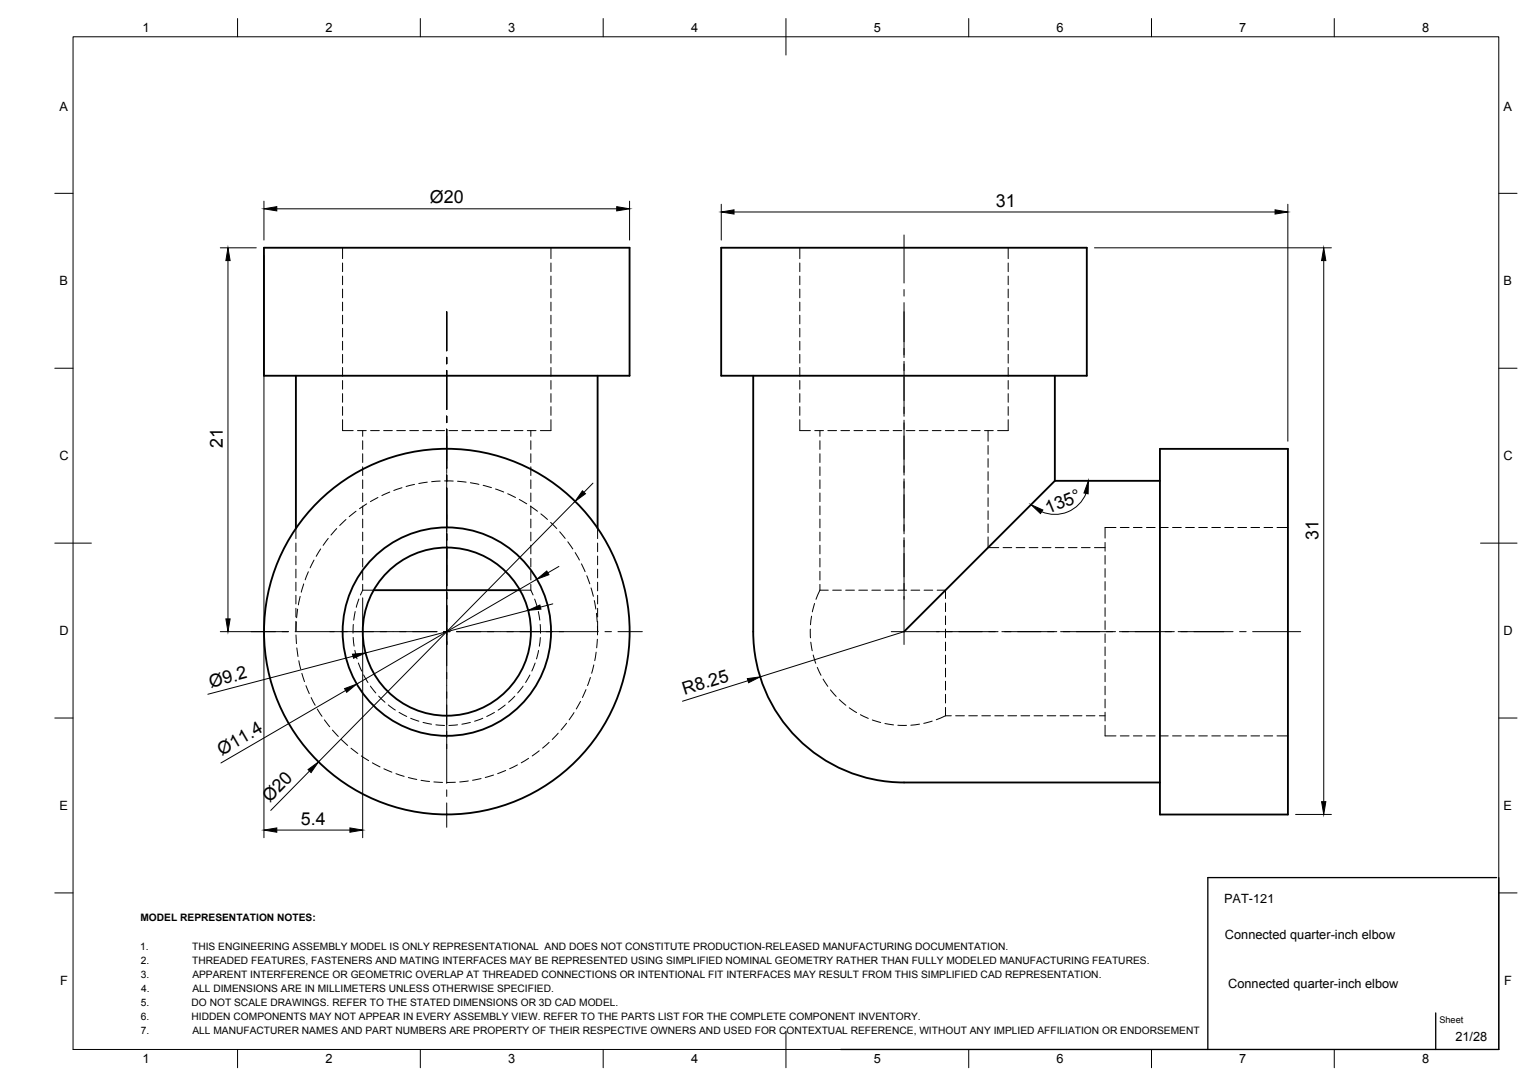
ISO-10303-21;
HEADER;
/* Generated by software containing ST-Developer
 * from STEP Tools, Inc. (www.steptools.com) 
 */

FILE_DESCRIPTION(
/* description */ ('Wall-mounted air drop station'),
/* implementation_level */ '2;1');

FILE_NAME(
/* name */ 'Connected quarter-inch elbow.step',
/* time_stamp */ '2026-10-28T22:16:19-07:00',
/* author */ (''),
/* organization */ (''),
/* preprocessor_version */ 'ST-DEVELOPER v20.2',
/* originating_system */ 'Autodesk Translation Framework v15.17.0.0',
/* authorisation */ '');

FILE_SCHEMA (('AUTOMOTIVE_DESIGN { 1 0 10303 214 3 1 1 }'));
ENDSEC;

DATA;
#10=MECHANICAL_DESIGN_GEOMETRIC_PRESENTATION_REPRESENTATION('',(#364),#10517);
#231=ELLIPSE('',#6687,0.650538238691624,0.46);
#232=ELLIPSE('',#6711,1.1667261889578,0.825);
#261=SPHERICAL_SURFACE('',#6691,0.513);
#262=SPHERICAL_SURFACE('',#6705,0.825);
#306=SHAPE_REPRESENTATION_RELATIONSHIP('SRR','None',#10663,#335);
#335=ADVANCED_BREP_SHAPE_REPRESENTATION('',(#391),#10507);
#364=STYLED_ITEM('',(#10888),#391);
#391=MANIFOLD_SOLID_BREP('Body1',#5905);
#505=FACE_BOUND('',#1465,.T.);
#506=FACE_BOUND('',#1468,.T.);
#507=FACE_BOUND('',#1472,.T.);
#508=FACE_BOUND('',#1476,.T.);
#509=FACE_BOUND('',#1479,.T.);
#510=FACE_BOUND('',#1481,.T.);
#511=FACE_BOUND('',#1484,.T.);
#676=PLANE('',#6697);
#677=PLANE('',#6704);
#678=PLANE('',#6713);
#679=PLANE('',#6717);
#680=PLANE('',#6718);
#681=PLANE('',#6723);
#1002=FACE_OUTER_BOUND('',#1463,.T.);
#1003=FACE_OUTER_BOUND('',#1464,.T.);
#1004=FACE_OUTER_BOUND('',#1466,.T.);
#1005=FACE_OUTER_BOUND('',#1467,.T.);
#1006=FACE_OUTER_BOUND('',#1469,.T.);
#1007=FACE_OUTER_BOUND('',#1470,.T.);
#1008=FACE_OUTER_BOUND('',#1471,.T.);
#1009=FACE_OUTER_BOUND('',#1473,.T.);
#1010=FACE_OUTER_BOUND('',#1474,.T.);
#1011=FACE_OUTER_BOUND('',#1475,.T.);
#1012=FACE_OUTER_BOUND('',#1477,.T.);
#1013=FACE_OUTER_BOUND('',#1478,.T.);
#1014=FACE_OUTER_BOUND('',#1480,.T.);
#1015=FACE_OUTER_BOUND('',#1482,.T.);
#1016=FACE_OUTER_BOUND('',#1483,.T.);
#1017=FACE_OUTER_BOUND('',#1485,.T.);
#1463=EDGE_LOOP('',(#4987,#4988,#4989,#4990,#4991,#4992));
#1464=EDGE_LOOP('',(#4993,#4994));
#1465=EDGE_LOOP('',(#4995,#4996,#4997,#4998));
#1466=EDGE_LOOP('',(#4999,#5000,#5001,#5002,#5003,#5004));
#1467=EDGE_LOOP('',(#5005));
#1468=EDGE_LOOP('',(#5006));
#1469=EDGE_LOOP('',(#5007,#5008,#5009,#5010));
#1470=EDGE_LOOP('',(#5011,#5012,#5013,#5014));
#1471=EDGE_LOOP('',(#5015));
#1472=EDGE_LOOP('',(#5016));
#1473=EDGE_LOOP('',(#5017,#5018,#5019,#5020));
#1474=EDGE_LOOP('',(#5021,#5022,#5023,#5024,#5025,#5026));
#1475=EDGE_LOOP('',(#5027));
#1476=EDGE_LOOP('',(#5028));
#1477=EDGE_LOOP('',(#5029,#5030,#5031,#5032));
#1478=EDGE_LOOP('',(#5033));
#1479=EDGE_LOOP('',(#5034));
#1480=EDGE_LOOP('',(#5035));
#1481=EDGE_LOOP('',(#5036));
#1482=EDGE_LOOP('',(#5037,#5038,#5039,#5040));
#1483=EDGE_LOOP('',(#5041));
#1484=EDGE_LOOP('',(#5042));
#1485=EDGE_LOOP('',(#5043,#5044,#5045,#5046,#5047,#5048));
#1906=LINE('',#9908,#2370);
#1907=LINE('',#9920,#2371);
#1908=LINE('',#9928,#2372);
#1909=LINE('',#9933,#2373);
#1910=LINE('',#9948,#2374);
#1911=LINE('',#9956,#2375);
#1912=LINE('',#9966,#2376);
#1913=LINE('',#9969,#2377);
#2370=VECTOR('',#8146,0.46);
#2371=VECTOR('',#8161,0.46);
#2372=VECTOR('',#8172,0.57);
#2373=VECTOR('',#8177,0.57);
#2374=VECTOR('',#8196,0.825);
#2375=VECTOR('',#8207,1.);
#2376=VECTOR('',#8220,1.);
#2377=VECTOR('',#8225,0.825);
#2701=CIRCLE('',#6688,0.46);
#2702=CIRCLE('',#6689,0.46);
#2703=CIRCLE('',#6690,0.46);
#2704=CIRCLE('',#6692,0.513);
#2705=CIRCLE('',#6693,0.46);
#2706=CIRCLE('',#6694,0.46);
#2707=CIRCLE('',#6696,0.46);
#2708=CIRCLE('',#6698,0.57);
#2709=CIRCLE('',#6700,0.57);
#2710=CIRCLE('',#6702,0.57);
#2711=CIRCLE('',#6703,0.57);
#2712=CIRCLE('',#6706,0.825);
#2713=CIRCLE('',#6707,0.825);
#2714=CIRCLE('',#6708,0.825);
#2715=CIRCLE('',#6709,0.825);
#2716=CIRCLE('',#6712,0.825);
#2717=CIRCLE('',#6714,1.);
#2718=CIRCLE('',#6716,1.);
#2719=CIRCLE('',#6719,1.);
#2720=CIRCLE('',#6720,0.825);
#2721=CIRCLE('',#6722,1.);
#3099=VERTEX_POINT('',#9902);
#3100=VERTEX_POINT('',#9903);
#3101=VERTEX_POINT('',#9905);
#3102=VERTEX_POINT('',#9907);
#3103=VERTEX_POINT('',#9912);
#3104=VERTEX_POINT('',#9913);
#3105=VERTEX_POINT('',#9915);
#3106=VERTEX_POINT('',#9919);
#3107=VERTEX_POINT('',#9923);
#3108=VERTEX_POINT('',#9926);
#3109=VERTEX_POINT('',#9930);
#3110=VERTEX_POINT('',#9932);
#3111=VERTEX_POINT('',#9937);
#3112=VERTEX_POINT('',#9938);
#3113=VERTEX_POINT('',#9940);
#3114=VERTEX_POINT('',#9942);
#3115=VERTEX_POINT('',#9947);
#3116=VERTEX_POINT('',#9951);
#3117=VERTEX_POINT('',#9954);
#3118=VERTEX_POINT('',#9959);
#3119=VERTEX_POINT('',#9961);
#3120=VERTEX_POINT('',#9964);
#3751=EDGE_CURVE('',#3099,#3100,#231,.T.);
#3752=EDGE_CURVE('',#3101,#3099,#2701,.T.);
#3753=EDGE_CURVE('',#3101,#3102,#1906,.T.);
#3754=EDGE_CURVE('',#3102,#3102,#2702,.T.);
#3755=EDGE_CURVE('',#3100,#3101,#2703,.T.);
#3756=EDGE_CURVE('',#3103,#3104,#2704,.T.);
#3757=EDGE_CURVE('',#3099,#3105,#2705,.T.);
#3758=EDGE_CURVE('',#3105,#3100,#2706,.T.);
#3759=EDGE_CURVE('',#3105,#3106,#1907,.T.);
#3760=EDGE_CURVE('',#3106,#3106,#2707,.T.);
#3761=EDGE_CURVE('',#3107,#3107,#2708,.T.);
#3762=EDGE_CURVE('',#3108,#3108,#2709,.T.);
#3763=EDGE_CURVE('',#3108,#3107,#1908,.T.);
#3764=EDGE_CURVE('',#3109,#3109,#2710,.T.);
#3765=EDGE_CURVE('',#3109,#3110,#1909,.T.);
#3766=EDGE_CURVE('',#3110,#3110,#2711,.T.);
#3767=EDGE_CURVE('',#3111,#3112,#2712,.T.);
#3768=EDGE_CURVE('',#3112,#3113,#2713,.T.);
#3769=EDGE_CURVE('',#3114,#3113,#2714,.T.);
#3770=EDGE_CURVE('',#3111,#3114,#2715,.T.);
#3771=EDGE_CURVE('',#3113,#3111,#232,.T.);
#3772=EDGE_CURVE('',#3112,#3115,#1910,.T.);
#3773=EDGE_CURVE('',#3115,#3115,#2716,.T.);
#3774=EDGE_CURVE('',#3116,#3116,#2717,.T.);
#3775=EDGE_CURVE('',#3117,#3117,#2718,.T.);
#3776=EDGE_CURVE('',#3117,#3116,#1911,.T.);
#3777=EDGE_CURVE('',#3118,#3118,#2719,.T.);
#3778=EDGE_CURVE('',#3119,#3119,#2720,.T.);
#3779=EDGE_CURVE('',#3120,#3120,#2721,.T.);
#3780=EDGE_CURVE('',#3120,#3118,#1912,.T.);
#3781=EDGE_CURVE('',#3119,#3114,#1913,.T.);
#4987=ORIENTED_EDGE('',*,*,#3751,.F.);
#4988=ORIENTED_EDGE('',*,*,#3752,.F.);
#4989=ORIENTED_EDGE('',*,*,#3753,.T.);
#4990=ORIENTED_EDGE('',*,*,#3754,.F.);
#4991=ORIENTED_EDGE('',*,*,#3753,.F.);
#4992=ORIENTED_EDGE('',*,*,#3755,.F.);
#4993=ORIENTED_EDGE('',*,*,#3756,.T.);
#4994=ORIENTED_EDGE('',*,*,#3756,.F.);
#4995=ORIENTED_EDGE('',*,*,#3755,.T.);
#4996=ORIENTED_EDGE('',*,*,#3752,.T.);
#4997=ORIENTED_EDGE('',*,*,#3757,.T.);
#4998=ORIENTED_EDGE('',*,*,#3758,.T.);
#4999=ORIENTED_EDGE('',*,*,#3751,.T.);
#5000=ORIENTED_EDGE('',*,*,#3758,.F.);
#5001=ORIENTED_EDGE('',*,*,#3759,.T.);
#5002=ORIENTED_EDGE('',*,*,#3760,.F.);
#5003=ORIENTED_EDGE('',*,*,#3759,.F.);
#5004=ORIENTED_EDGE('',*,*,#3757,.F.);
#5005=ORIENTED_EDGE('',*,*,#3761,.F.);
#5006=ORIENTED_EDGE('',*,*,#3754,.T.);
#5007=ORIENTED_EDGE('',*,*,#3762,.F.);
#5008=ORIENTED_EDGE('',*,*,#3763,.T.);
#5009=ORIENTED_EDGE('',*,*,#3761,.T.);
#5010=ORIENTED_EDGE('',*,*,#3763,.F.);
#5011=ORIENTED_EDGE('',*,*,#3764,.F.);
#5012=ORIENTED_EDGE('',*,*,#3765,.T.);
#5013=ORIENTED_EDGE('',*,*,#3766,.F.);
#5014=ORIENTED_EDGE('',*,*,#3765,.F.);
#5015=ORIENTED_EDGE('',*,*,#3764,.T.);
#5016=ORIENTED_EDGE('',*,*,#3760,.T.);
#5017=ORIENTED_EDGE('',*,*,#3767,.T.);
#5018=ORIENTED_EDGE('',*,*,#3768,.T.);
#5019=ORIENTED_EDGE('',*,*,#3769,.F.);
#5020=ORIENTED_EDGE('',*,*,#3770,.F.);
#5021=ORIENTED_EDGE('',*,*,#3771,.F.);
#5022=ORIENTED_EDGE('',*,*,#3768,.F.);
#5023=ORIENTED_EDGE('',*,*,#3772,.T.);
#5024=ORIENTED_EDGE('',*,*,#3773,.T.);
#5025=ORIENTED_EDGE('',*,*,#3772,.F.);
#5026=ORIENTED_EDGE('',*,*,#3767,.F.);
#5027=ORIENTED_EDGE('',*,*,#3774,.F.);
#5028=ORIENTED_EDGE('',*,*,#3762,.T.);
#5029=ORIENTED_EDGE('',*,*,#3775,.F.);
#5030=ORIENTED_EDGE('',*,*,#3776,.T.);
#5031=ORIENTED_EDGE('',*,*,#3774,.T.);
#5032=ORIENTED_EDGE('',*,*,#3776,.F.);
#5033=ORIENTED_EDGE('',*,*,#3775,.T.);
#5034=ORIENTED_EDGE('',*,*,#3773,.F.);
#5035=ORIENTED_EDGE('',*,*,#3777,.F.);
#5036=ORIENTED_EDGE('',*,*,#3778,.T.);
#5037=ORIENTED_EDGE('',*,*,#3779,.F.);
#5038=ORIENTED_EDGE('',*,*,#3780,.T.);
#5039=ORIENTED_EDGE('',*,*,#3777,.T.);
#5040=ORIENTED_EDGE('',*,*,#3780,.F.);
#5041=ORIENTED_EDGE('',*,*,#3779,.T.);
#5042=ORIENTED_EDGE('',*,*,#3766,.T.);
#5043=ORIENTED_EDGE('',*,*,#3778,.F.);
#5044=ORIENTED_EDGE('',*,*,#3781,.T.);
#5045=ORIENTED_EDGE('',*,*,#3769,.T.);
#5046=ORIENTED_EDGE('',*,*,#3771,.T.);
#5047=ORIENTED_EDGE('',*,*,#3770,.T.);
#5048=ORIENTED_EDGE('',*,*,#3781,.F.);
#5509=CYLINDRICAL_SURFACE('',#6686,0.46);
#5510=CYLINDRICAL_SURFACE('',#6695,0.46);
#5511=CYLINDRICAL_SURFACE('',#6699,0.57);
#5512=CYLINDRICAL_SURFACE('',#6701,0.57);
#5513=CYLINDRICAL_SURFACE('',#6710,0.825);
#5514=CYLINDRICAL_SURFACE('',#6715,1.);
#5515=CYLINDRICAL_SURFACE('',#6721,1.);
#5516=CYLINDRICAL_SURFACE('',#6724,0.825);
#5775=ADVANCED_FACE('',(#1002),#5509,.F.);
#5776=ADVANCED_FACE('',(#1003,#505),#261,.F.);
#5777=ADVANCED_FACE('',(#1004),#5510,.F.);
#5778=ADVANCED_FACE('',(#1005,#506),#676,.F.);
#5779=ADVANCED_FACE('',(#1006),#5511,.F.);
#5780=ADVANCED_FACE('',(#1007),#5512,.F.);
#5781=ADVANCED_FACE('',(#1008,#507),#677,.F.);
#5782=ADVANCED_FACE('',(#1009),#262,.T.);
#5783=ADVANCED_FACE('',(#1010),#5513,.T.);
#5784=ADVANCED_FACE('',(#1011,#508),#678,.T.);
#5785=ADVANCED_FACE('',(#1012),#5514,.T.);
#5786=ADVANCED_FACE('',(#1013,#509),#679,.T.);
#5787=ADVANCED_FACE('',(#1014,#510),#680,.T.);
#5788=ADVANCED_FACE('',(#1015),#5515,.T.);
#5789=ADVANCED_FACE('',(#1016,#511),#681,.T.);
#5790=ADVANCED_FACE('',(#1017),#5516,.T.);
#5905=CLOSED_SHELL('',(#5775,#5776,#5777,#5778,#5779,#5780,#5781,#5782,
#5783,#5784,#5785,#5786,#5787,#5788,#5789,#5790));
#6685=AXIS2_PLACEMENT_3D('',#9900,#8138,#8139);
#6686=AXIS2_PLACEMENT_3D('',#9901,#8140,#8141);
#6687=AXIS2_PLACEMENT_3D('',#9904,#8142,#8143);
#6688=AXIS2_PLACEMENT_3D('',#9906,#8144,#8145);
#6689=AXIS2_PLACEMENT_3D('',#9909,#8147,#8148);
#6690=AXIS2_PLACEMENT_3D('',#9910,#8149,#8150);
#6691=AXIS2_PLACEMENT_3D('',#9911,#8151,#8152);
#6692=AXIS2_PLACEMENT_3D('',#9914,#8153,#8154);
#6693=AXIS2_PLACEMENT_3D('',#9916,#8155,#8156);
#6694=AXIS2_PLACEMENT_3D('',#9917,#8157,#8158);
#6695=AXIS2_PLACEMENT_3D('',#9918,#8159,#8160);
#6696=AXIS2_PLACEMENT_3D('',#9921,#8162,#8163);
#6697=AXIS2_PLACEMENT_3D('',#9922,#8164,#8165);
#6698=AXIS2_PLACEMENT_3D('',#9924,#8166,#8167);
#6699=AXIS2_PLACEMENT_3D('',#9925,#8168,#8169);
#6700=AXIS2_PLACEMENT_3D('',#9927,#8170,#8171);
#6701=AXIS2_PLACEMENT_3D('',#9929,#8173,#8174);
#6702=AXIS2_PLACEMENT_3D('',#9931,#8175,#8176);
#6703=AXIS2_PLACEMENT_3D('',#9934,#8178,#8179);
#6704=AXIS2_PLACEMENT_3D('',#9935,#8180,#8181);
#6705=AXIS2_PLACEMENT_3D('',#9936,#8182,#8183);
#6706=AXIS2_PLACEMENT_3D('',#9939,#8184,#8185);
#6707=AXIS2_PLACEMENT_3D('',#9941,#8186,#8187);
#6708=AXIS2_PLACEMENT_3D('',#9943,#8188,#8189);
#6709=AXIS2_PLACEMENT_3D('',#9944,#8190,#8191);
#6710=AXIS2_PLACEMENT_3D('',#9945,#8192,#8193);
#6711=AXIS2_PLACEMENT_3D('',#9946,#8194,#8195);
#6712=AXIS2_PLACEMENT_3D('',#9949,#8197,#8198);
#6713=AXIS2_PLACEMENT_3D('',#9950,#8199,#8200);
#6714=AXIS2_PLACEMENT_3D('',#9952,#8201,#8202);
#6715=AXIS2_PLACEMENT_3D('',#9953,#8203,#8204);
#6716=AXIS2_PLACEMENT_3D('',#9955,#8205,#8206);
#6717=AXIS2_PLACEMENT_3D('',#9957,#8208,#8209);
#6718=AXIS2_PLACEMENT_3D('',#9958,#8210,#8211);
#6719=AXIS2_PLACEMENT_3D('',#9960,#8212,#8213);
#6720=AXIS2_PLACEMENT_3D('',#9962,#8214,#8215);
#6721=AXIS2_PLACEMENT_3D('',#9963,#8216,#8217);
#6722=AXIS2_PLACEMENT_3D('',#9965,#8218,#8219);
#6723=AXIS2_PLACEMENT_3D('',#9967,#8221,#8222);
#6724=AXIS2_PLACEMENT_3D('',#9968,#8223,#8224);
#8138=DIRECTION('axis',(0.,0.,1.));
#8139=DIRECTION('refdir',(1.,0.,0.));
#8140=DIRECTION('center_axis',(0.,1.,0.));
#8141=DIRECTION('ref_axis',(1.,0.,0.));
#8142=DIRECTION('center_axis',(-0.707106781186548,0.707106781186548,0.));
#8143=DIRECTION('ref_axis',(0.707106781186548,0.707106781186548,0.));
#8144=DIRECTION('center_axis',(0.,1.,0.));
#8145=DIRECTION('ref_axis',(1.,-6.03382078600629E-17,0.));
#8146=DIRECTION('',(0.,1.,0.));
#8147=DIRECTION('center_axis',(0.,-1.,0.));
#8148=DIRECTION('ref_axis',(1.,0.,0.));
#8149=DIRECTION('center_axis',(0.,1.,0.));
#8150=DIRECTION('ref_axis',(1.,-6.03382078600629E-17,0.));
#8151=DIRECTION('center_axis',(6.12323399573677E-17,0.,1.));
#8152=DIRECTION('ref_axis',(1.,0.,0.));
#8153=DIRECTION('center_axis',(-1.22464679914735E-16,1.,0.));
#8154=DIRECTION('ref_axis',(-1.,-1.22464679914735E-16,0.));
#8155=DIRECTION('center_axis',(1.,0.,0.));
#8156=DIRECTION('ref_axis',(-6.03382078600629E-17,0.,-1.));
#8157=DIRECTION('center_axis',(1.,0.,0.));
#8158=DIRECTION('ref_axis',(-6.03382078600629E-17,0.,-1.));
#8159=DIRECTION('center_axis',(1.,0.,0.));
#8160=DIRECTION('ref_axis',(0.,0.,-1.));
#8161=DIRECTION('',(1.,0.,0.));
#8162=DIRECTION('center_axis',(-1.,0.,0.));
#8163=DIRECTION('ref_axis',(0.,0.,-1.));
#8164=DIRECTION('center_axis',(0.,-1.,0.));
#8165=DIRECTION('ref_axis',(0.,0.,-1.));
#8166=DIRECTION('center_axis',(0.,-1.,0.));
#8167=DIRECTION('ref_axis',(1.,0.,0.));
#8168=DIRECTION('center_axis',(0.,-1.,0.));
#8169=DIRECTION('ref_axis',(1.,0.,0.));
#8170=DIRECTION('center_axis',(0.,-1.,0.));
#8171=DIRECTION('ref_axis',(1.,0.,0.));
#8172=DIRECTION('',(0.,-1.,0.));
#8173=DIRECTION('center_axis',(1.,0.,0.));
#8174=DIRECTION('ref_axis',(0.,1.,0.));
#8175=DIRECTION('center_axis',(1.,0.,0.));
#8176=DIRECTION('ref_axis',(0.,0.,-1.));
#8177=DIRECTION('',(1.,0.,0.));
#8178=DIRECTION('center_axis',(-1.,0.,0.));
#8179=DIRECTION('ref_axis',(0.,1.,0.));
#8180=DIRECTION('center_axis',(-1.,0.,0.));
#8181=DIRECTION('ref_axis',(0.,0.,1.));
#8182=DIRECTION('center_axis',(6.12323399573677E-17,0.,1.));
#8183=DIRECTION('ref_axis',(1.,0.,0.));
#8184=DIRECTION('center_axis',(0.,-1.,0.));
#8185=DIRECTION('ref_axis',(1.,0.,0.));
#8186=DIRECTION('center_axis',(0.,-1.,0.));
#8187=DIRECTION('ref_axis',(1.,0.,0.));
#8188=DIRECTION('center_axis',(1.,0.,0.));
#8189=DIRECTION('ref_axis',(0.,0.,-1.));
#8190=DIRECTION('center_axis',(1.,0.,0.));
#8191=DIRECTION('ref_axis',(0.,0.,-1.));
#8192=DIRECTION('center_axis',(0.,-1.,0.));
#8193=DIRECTION('ref_axis',(1.,0.,0.));
#8194=DIRECTION('center_axis',(0.707106781186548,-0.707106781186548,0.));
#8195=DIRECTION('ref_axis',(0.707106781186548,0.707106781186547,0.));
#8196=DIRECTION('',(0.,1.,0.));
#8197=DIRECTION('center_axis',(0.,-1.,0.));
#8198=DIRECTION('ref_axis',(1.,0.,0.));
#8199=DIRECTION('center_axis',(0.,1.,0.));
#8200=DIRECTION('ref_axis',(0.,0.,1.));
#8201=DIRECTION('center_axis',(0.,-1.,0.));
#8202=DIRECTION('ref_axis',(1.,0.,0.));
#8203=DIRECTION('center_axis',(0.,-1.,0.));
#8204=DIRECTION('ref_axis',(1.,0.,0.));
#8205=DIRECTION('center_axis',(0.,-1.,0.));
#8206=DIRECTION('ref_axis',(1.,0.,0.));
#8207=DIRECTION('',(0.,1.,0.));
#8208=DIRECTION('center_axis',(0.,-1.,0.));
#8209=DIRECTION('ref_axis',(0.,0.,-1.));
#8210=DIRECTION('center_axis',(-1.,0.,0.));
#8211=DIRECTION('ref_axis',(0.,0.,1.));
#8212=DIRECTION('center_axis',(1.,0.,0.));
#8213=DIRECTION('ref_axis',(0.,0.,-1.));
#8214=DIRECTION('center_axis',(1.,0.,0.));
#8215=DIRECTION('ref_axis',(0.,0.,-1.));
#8216=DIRECTION('center_axis',(1.,0.,0.));
#8217=DIRECTION('ref_axis',(0.,1.,0.));
#8218=DIRECTION('center_axis',(1.,0.,0.));
#8219=DIRECTION('ref_axis',(0.,0.,-1.));
#8220=DIRECTION('',(-1.,0.,0.));
#8221=DIRECTION('center_axis',(1.,0.,0.));
#8222=DIRECTION('ref_axis',(0.,0.,-1.));
#8223=DIRECTION('center_axis',(1.,0.,0.));
#8224=DIRECTION('ref_axis',(0.,1.,0.));
#8225=DIRECTION('',(-1.,0.,0.));
#9900=CARTESIAN_POINT('',(0.,0.,0.));
#9901=CARTESIAN_POINT('Origin',(0.,-0.1,0.));
#9902=CARTESIAN_POINT('',(0.227088088635226,0.227088088635225,0.400038748123229));
#9903=CARTESIAN_POINT('',(0.227088088635226,0.227088088635225,-0.400038748123229));
#9904=CARTESIAN_POINT('Origin',(0.,0.,0.));
#9905=CARTESIAN_POINT('',(-0.46,0.227088088635226,5.63337527607782E-17));
#9906=CARTESIAN_POINT('Origin',(0.,0.227088088635226,0.));
#9907=CARTESIAN_POINT('',(-0.46,1.1,-5.63337527607782E-17));
#9908=CARTESIAN_POINT('',(-0.46,-0.1,5.63337527607782E-17));
#9909=CARTESIAN_POINT('Origin',(0.,1.1,0.));
#9910=CARTESIAN_POINT('Origin',(0.,0.227088088635226,0.));
#9911=CARTESIAN_POINT('Origin',(0.,0.,0.));
#9912=CARTESIAN_POINT('',(-3.14121903981296E-17,-3.84688384252766E-33,-0.513));
#9913=CARTESIAN_POINT('',(-3.14121903981296E-17,-3.84688384252766E-33,0.513));
#9914=CARTESIAN_POINT('Origin',(0.,0.,0.));
#9915=CARTESIAN_POINT('',(0.227088088635226,-5.63337527607782E-17,0.46));
#9916=CARTESIAN_POINT('Origin',(0.227088088635226,0.,0.));
#9917=CARTESIAN_POINT('Origin',(0.227088088635226,0.,0.));
#9918=CARTESIAN_POINT('Origin',(-0.1,0.,0.));
#9919=CARTESIAN_POINT('',(1.1,5.63337527607782E-17,0.46));
#9920=CARTESIAN_POINT('',(-0.1,-5.63337527607782E-17,0.46));
#9921=CARTESIAN_POINT('Origin',(1.1,0.,0.));
#9922=CARTESIAN_POINT('Origin',(0.,1.1,0.));
#9923=CARTESIAN_POINT('',(-0.57,1.1,-6.98048675513991E-17));
#9924=CARTESIAN_POINT('Origin',(0.,1.1,0.));
#9925=CARTESIAN_POINT('Origin',(0.,1.65,0.));
#9926=CARTESIAN_POINT('',(-0.57,2.1,-6.98048675513991E-17));
#9927=CARTESIAN_POINT('Origin',(0.,2.1,0.));
#9928=CARTESIAN_POINT('',(-0.57,1.65,-6.98048675513991E-17));
#9929=CARTESIAN_POINT('Origin',(1.65,0.,0.));
#9930=CARTESIAN_POINT('',(1.1,-0.57,-6.98048675513991E-17));
#9931=CARTESIAN_POINT('Origin',(1.1,0.,0.));
#9932=CARTESIAN_POINT('',(2.1,-0.57,6.98048675513991E-17));
#9933=CARTESIAN_POINT('',(1.65,-0.57,-6.98048675513991E-17));
#9934=CARTESIAN_POINT('Origin',(2.1,0.,0.));
#9935=CARTESIAN_POINT('Origin',(1.1,0.57,0.));
#9936=CARTESIAN_POINT('Origin',(0.,0.,0.));
#9937=CARTESIAN_POINT('',(0.,0.,0.825));
#9938=CARTESIAN_POINT('',(-0.825,0.,-1.01033360929657E-16));
#9939=CARTESIAN_POINT('Origin',(0.,0.,0.));
#9940=CARTESIAN_POINT('',(0.,0.,-0.825));
#9941=CARTESIAN_POINT('Origin',(0.,0.,0.));
#9942=CARTESIAN_POINT('',(0.,-0.825,-1.01033360929657E-16));
#9943=CARTESIAN_POINT('Origin',(0.,0.,0.));
#9944=CARTESIAN_POINT('Origin',(0.,0.,0.));
#9945=CARTESIAN_POINT('Origin',(0.,0.7,0.));
#9946=CARTESIAN_POINT('Origin',(0.,0.,0.));
#9947=CARTESIAN_POINT('',(-0.825,1.4,-1.01033360929657E-16));
#9948=CARTESIAN_POINT('',(-0.825,0.7,-1.01033360929657E-16));
#9949=CARTESIAN_POINT('Origin',(0.,1.4,0.));
#9950=CARTESIAN_POINT('Origin',(1.,2.1,0.));
#9951=CARTESIAN_POINT('',(-1.,2.1,-1.22464679914735E-16));
#9952=CARTESIAN_POINT('Origin',(0.,2.1,0.));
#9953=CARTESIAN_POINT('Origin',(0.,1.75,0.));
#9954=CARTESIAN_POINT('',(-1.,1.4,-1.22464679914735E-16));
#9955=CARTESIAN_POINT('Origin',(0.,1.4,0.));
#9956=CARTESIAN_POINT('',(-1.,1.75,-1.22464679914735E-16));
#9957=CARTESIAN_POINT('Origin',(0.825,1.4,0.));
#9958=CARTESIAN_POINT('Origin',(1.4,1.,0.));
#9959=CARTESIAN_POINT('',(1.4,-1.,-1.22464679914735E-16));
#9960=CARTESIAN_POINT('Origin',(1.4,0.,0.));
#9961=CARTESIAN_POINT('',(1.4,-0.825,-1.01033360929657E-16));
#9962=CARTESIAN_POINT('Origin',(1.4,0.,0.));
#9963=CARTESIAN_POINT('Origin',(1.75,0.,0.));
#9964=CARTESIAN_POINT('',(2.1,-1.,-1.22464679914735E-16));
#9965=CARTESIAN_POINT('Origin',(2.1,0.,0.));
#9966=CARTESIAN_POINT('',(1.75,-1.,-1.22464679914735E-16));
#9967=CARTESIAN_POINT('Origin',(2.1,0.,0.));
#9968=CARTESIAN_POINT('Origin',(0.7,0.,0.));
#9969=CARTESIAN_POINT('',(0.7,-0.825,-1.01033360929657E-16));
#10474=UNCERTAINTY_MEASURE_WITH_UNIT(LENGTH_MEASURE(0.001),#10518,
'DISTANCE_ACCURACY_VALUE',
'Maximum model space distance between geometric entities at asserted c
onnectivities');
#10484=UNCERTAINTY_MEASURE_WITH_UNIT(LENGTH_MEASURE(0.001),#10518,
'DISTANCE_ACCURACY_VALUE',
'Maximum model space distance between geometric entities at asserted c
onnectivities');
#10507=(
GEOMETRIC_REPRESENTATION_CONTEXT(3)
GLOBAL_UNCERTAINTY_ASSIGNED_CONTEXT((#10474))
GLOBAL_UNIT_ASSIGNED_CONTEXT((#10518,#10520,#10521))
REPRESENTATION_CONTEXT('','3D')
);
#10517=(
GEOMETRIC_REPRESENTATION_CONTEXT(3)
GLOBAL_UNCERTAINTY_ASSIGNED_CONTEXT((#10484))
GLOBAL_UNIT_ASSIGNED_CONTEXT((#10518,#10520,#10521))
REPRESENTATION_CONTEXT('','3D')
);
#10518=(
LENGTH_UNIT()
NAMED_UNIT(*)
SI_UNIT(.CENTI.,.METRE.)
);
#10520=(
NAMED_UNIT(*)
PLANE_ANGLE_UNIT()
SI_UNIT($,.RADIAN.)
);
#10521=(
NAMED_UNIT(*)
SI_UNIT($,.STERADIAN.)
SOLID_ANGLE_UNIT()
);
#10544=SHAPE_DEFINITION_REPRESENTATION(#10576,#10663);
#10576=PRODUCT_DEFINITION_SHAPE('',$,#10696);
#10663=SHAPE_REPRESENTATION('',(#6685),#10507);
#10673=PRODUCT_DEFINITION_CONTEXT('part definition',#10771,'design');
#10696=PRODUCT_DEFINITION('Connected quarter-inch elbow',
'Connected quarter-inch elbow',#10728,#10673);
#10728=PRODUCT_DEFINITION_FORMATION('',$,#10795);
#10771=APPLICATION_CONTEXT(
'Core Data for Automotive Mechanical Design Process');
#10772=PRODUCT_CONTEXT('part definition',#10771,'mechanical');
#10795=PRODUCT('Connected quarter-inch elbow',
'Connected quarter-inch elbow','Connected quarter-inch elbow',(#10772));
#10882=COLOUR_RGB('Off White',0.89,0.88,0.83);
#10883=FILL_AREA_STYLE_COLOUR('',#10882);
#10884=FILL_AREA_STYLE('',(#10883));
#10885=SURFACE_STYLE_FILL_AREA(#10884);
#10886=SURFACE_SIDE_STYLE('',(#10885));
#10887=SURFACE_STYLE_USAGE(.BOTH.,#10886);
#10888=PRESENTATION_STYLE_ASSIGNMENT((#10887));
ENDSEC;
END-ISO-10303-21;
